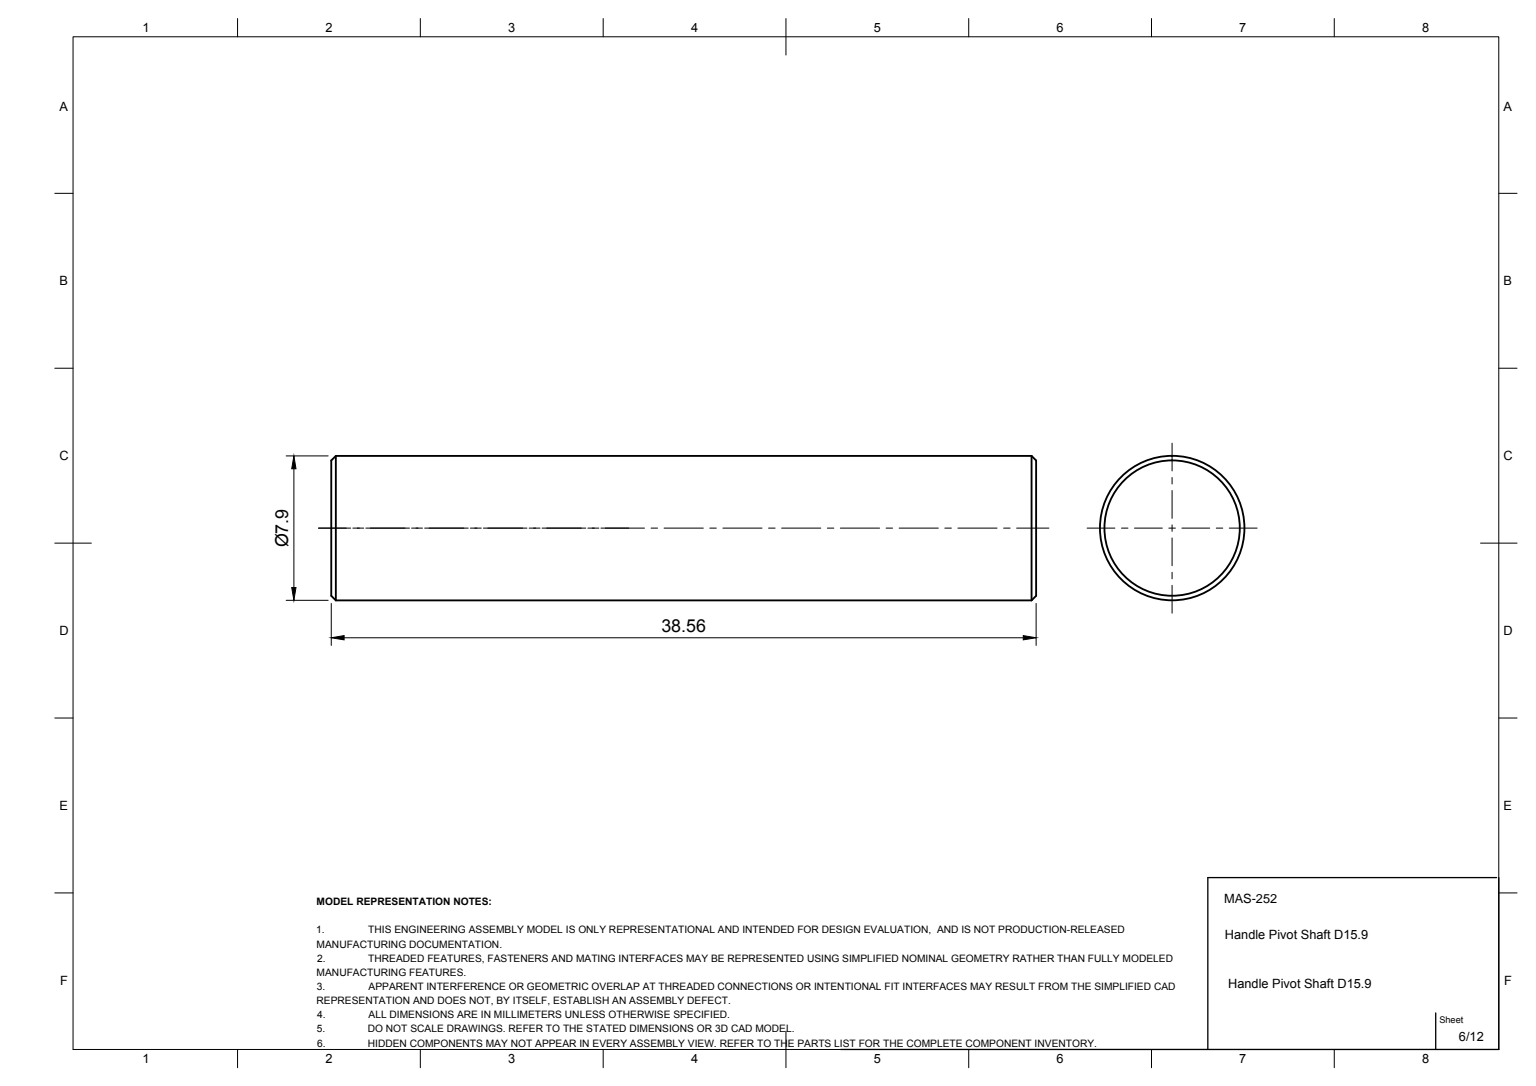
ISO-10303-21;
HEADER;
FILE_DESCRIPTION((''),'2;1');
FILE_NAME('Handle Pivot Shaft D15.9.step','2026-10-06T07:01:46+05:00',(''),(''),'','','');
FILE_SCHEMA (('AUTOMOTIVE_DESIGN { 1 0 10303 214 3 1 1 }'));
ENDSEC;
DATA;
#10=MECHANICAL_DESIGN_GEOMETRIC_PRESENTATION_REPRESENTATION('',(#141),#11396);
#95=CONICAL_SURFACE('',#6218,3.825,0.785398163397448) ;
#96=CONICAL_SURFACE('',#6222,3.825,0.785398163397448) ;
#111=SHAPE_REPRESENTATION_RELATIONSHIP('SRR','None',#11458,#126) ;
#126=ADVANCED_BREP_SHAPE_REPRESENTATION('',(#156),#11384) ;
#141=STYLED_ITEM('',(#11542),#156) ;
#156=MANIFOLD_SOLID_BREP('Handle Pivot Shaft D15.9',#5572) ;
#460=PLANE('',#6216) ;
#461=PLANE('',#6224) ;
#752=FACE_OUTER_BOUND('',#1114,.T.) ;
#753=FACE_OUTER_BOUND('',#1115,.T.) ;
#754=FACE_OUTER_BOUND('',#1116,.T.) ;
#755=FACE_OUTER_BOUND('',#1117,.T.) ;
#756=FACE_OUTER_BOUND('',#1118,.T.) ;
#1114=EDGE_LOOP('',(#4712)) ;
#1115=EDGE_LOOP('',(#4713,#4714,#4715,#4716)) ;
#1116=EDGE_LOOP('',(#4717,#4718,#4719,#4720)) ;
#1117=EDGE_LOOP('',(#4721,#4722,#4723,#4724)) ;
#1118=EDGE_LOOP('',(#4725)) ;
#1495=LINE('',#10802,#1878) ;
#1496=LINE('',#10806,#1879) ;
#1497=LINE('',#10810,#1880) ;
#1878=VECTOR('',#7629,3.825) ;
#1879=VECTOR('',#7634,3.95) ;
#1880=VECTOR('',#7639,3.825) ;
#2194=CIRCLE('',#6217,3.7) ;
#2195=CIRCLE('',#6219,3.95) ;
#2196=CIRCLE('',#6221,3.95) ;
#2197=CIRCLE('',#6223,3.7) ;
#2623=VERTEX_POINT('',#10797) ;
#2624=VERTEX_POINT('',#10800) ;
#2625=VERTEX_POINT('',#10804) ;
#2626=VERTEX_POINT('',#10808) ;
#3338=EDGE_CURVE('',#2623,#2623,#2194,.T.) ;
#3339=EDGE_CURVE('',#2624,#2624,#2195,.T.) ;
#3340=EDGE_CURVE('',#2624,#2623,#1495,.T.) ;
#3341=EDGE_CURVE('',#2625,#2625,#2196,.T.) ;
#3342=EDGE_CURVE('',#2625,#2624,#1496,.T.) ;
#3343=EDGE_CURVE('',#2626,#2626,#2197,.T.) ;
#3344=EDGE_CURVE('',#2626,#2625,#1497,.T.) ;
#4712=ORIENTED_EDGE('',*,*,#3338,.F.) ;
#4713=ORIENTED_EDGE('',*,*,#3339,.F.) ;
#4714=ORIENTED_EDGE('',*,*,#3340,.T.) ;
#4715=ORIENTED_EDGE('',*,*,#3338,.T.) ;
#4716=ORIENTED_EDGE('',*,*,#3340,.F.) ;
#4717=ORIENTED_EDGE('',*,*,#3341,.F.) ;
#4718=ORIENTED_EDGE('',*,*,#3342,.T.) ;
#4719=ORIENTED_EDGE('',*,*,#3339,.T.) ;
#4720=ORIENTED_EDGE('',*,*,#3342,.F.) ;
#4721=ORIENTED_EDGE('',*,*,#3343,.F.) ;
#4722=ORIENTED_EDGE('',*,*,#3344,.T.) ;
#4723=ORIENTED_EDGE('',*,*,#3341,.T.) ;
#4724=ORIENTED_EDGE('',*,*,#3344,.F.) ;
#4725=ORIENTED_EDGE('',*,*,#3343,.T.) ;
#5204=CYLINDRICAL_SURFACE('',#6220,3.95) ;
#5477=ADVANCED_FACE('',(#752),#460,.T.) ;
#5478=ADVANCED_FACE('',(#753),#95,.T.) ;
#5479=ADVANCED_FACE('',(#754),#5204,.T.) ;
#5480=ADVANCED_FACE('',(#755),#96,.T.) ;
#5481=ADVANCED_FACE('',(#756),#461,.T.) ;
#5572=CLOSED_SHELL('',(#5477,#5478,#5479,#5480,#5481)) ;
#6215=AXIS2_PLACEMENT_3D('',#10795,#7619,#7620) ;
#6216=AXIS2_PLACEMENT_3D('',#10796,#7621,#7622) ;
#6217=AXIS2_PLACEMENT_3D('',#10798,#7623,#7624) ;
#6218=AXIS2_PLACEMENT_3D('',#10799,#7625,#7626) ;
#6219=AXIS2_PLACEMENT_3D('',#10801,#7627,#7628) ;
#6220=AXIS2_PLACEMENT_3D('',#10803,#7630,#7631) ;
#6221=AXIS2_PLACEMENT_3D('',#10805,#7632,#7633) ;
#6222=AXIS2_PLACEMENT_3D('',#10807,#7635,#7636) ;
#6223=AXIS2_PLACEMENT_3D('',#10809,#7637,#7638) ;
#6224=AXIS2_PLACEMENT_3D('',#10811,#7640,#7641) ;
#7619=DIRECTION('axis',(0.,0.,1.)) ;
#7620=DIRECTION('refdir',(1.,0.,0.)) ;
#7621=DIRECTION('center_axis',(-1.,0.,0.)) ;
#7622=DIRECTION('ref_axis',(0.,0.,1.)) ;
#7623=DIRECTION('center_axis',(1.,0.,0.)) ;
#7624=DIRECTION('ref_axis',(0.,0.,-1.)) ;
#7625=DIRECTION('center_axis',(1.,0.,0.)) ;
#7626=DIRECTION('ref_axis',(0.,1.,0.)) ;
#7627=DIRECTION('center_axis',(1.,0.,0.)) ;
#7628=DIRECTION('ref_axis',(0.,0.,-1.)) ;
#7629=DIRECTION('',(-0.707106781186548,0.707106781186548,8.65956056235493E-17)) ;
#7630=DIRECTION('center_axis',(1.,0.,0.)) ;
#7631=DIRECTION('ref_axis',(0.,1.,0.)) ;
#7632=DIRECTION('center_axis',(1.,0.,0.)) ;
#7633=DIRECTION('ref_axis',(0.,0.,-1.)) ;
#7634=DIRECTION('',(-1.,0.,0.)) ;
#7635=DIRECTION('center_axis',(-1.,0.,0.)) ;
#7636=DIRECTION('ref_axis',(0.,1.,0.)) ;
#7637=DIRECTION('center_axis',(1.,0.,0.)) ;
#7638=DIRECTION('ref_axis',(0.,0.,-1.)) ;
#7639=DIRECTION('',(-0.707106781186548,-0.707106781186548,-8.65956056235493E-17)) ;
#7640=DIRECTION('center_axis',(1.,0.,0.)) ;
#7641=DIRECTION('ref_axis',(0.,0.,-1.)) ;
#10795=CARTESIAN_POINT('',(0.,0.,0.)) ;
#10796=CARTESIAN_POINT('Origin',(-27.15,21.265,27.14)) ;
#10797=CARTESIAN_POINT('',(-27.15,13.865,27.14)) ;
#10798=CARTESIAN_POINT('Origin',(-27.15,17.565,27.14)) ;
#10799=CARTESIAN_POINT('Origin',(-27.025,17.565,27.14)) ;
#10800=CARTESIAN_POINT('',(-26.9,13.615,27.14)) ;
#10801=CARTESIAN_POINT('Origin',(-26.9,17.565,27.14)) ;
#10802=CARTESIAN_POINT('',(-27.025,13.74,27.14)) ;
#10803=CARTESIAN_POINT('Origin',(-7.87,17.565,27.14)) ;
#10804=CARTESIAN_POINT('',(11.16,13.615,27.14)) ;
#10805=CARTESIAN_POINT('Origin',(11.16,17.565,27.14)) ;
#10806=CARTESIAN_POINT('',(-7.87,13.615,27.14)) ;
#10807=CARTESIAN_POINT('Origin',(11.285,17.565,27.14)) ;
#10808=CARTESIAN_POINT('',(11.41,13.865,27.14)) ;
#10809=CARTESIAN_POINT('Origin',(11.41,17.565,27.14)) ;
#10810=CARTESIAN_POINT('',(11.285,13.74,27.14)) ;
#10811=CARTESIAN_POINT('Origin',(11.41,17.565,27.14)) ;
#11367=UNCERTAINTY_MEASURE_WITH_UNIT(LENGTH_MEASURE(0.01),#11397,
'DISTANCE_ACCURACY_VALUE',
'Maximum model space distance between geometric entities at asserted c
onnectivities') ;
#11379=UNCERTAINTY_MEASURE_WITH_UNIT(LENGTH_MEASURE(0.01),#11397,
'DISTANCE_ACCURACY_VALUE',
'Maximum model space distance between geometric entities at asserted c
onnectivities') ;
#11384=(
GEOMETRIC_REPRESENTATION_CONTEXT(3)
GLOBAL_UNCERTAINTY_ASSIGNED_CONTEXT((#11367))
GLOBAL_UNIT_ASSIGNED_CONTEXT((#11397,#11399,#11400))
REPRESENTATION_CONTEXT('','3D')
) ;
#11396=(
GEOMETRIC_REPRESENTATION_CONTEXT(3)
GLOBAL_UNCERTAINTY_ASSIGNED_CONTEXT((#11379))
GLOBAL_UNIT_ASSIGNED_CONTEXT((#11397,#11399,#11400))
REPRESENTATION_CONTEXT('','3D')
) ;
#11397=(
LENGTH_UNIT()
NAMED_UNIT(*)
SI_UNIT(.MILLI.,.METRE.)
) ;
#11399=(
NAMED_UNIT(*)
PLANE_ANGLE_UNIT()
SI_UNIT($,.RADIAN.)
) ;
#11400=(
NAMED_UNIT(*)
SI_UNIT($,.STERADIAN.)
SOLID_ANGLE_UNIT()
) ;
#11405=SHAPE_DEFINITION_REPRESENTATION(#11421,#11458) ;
#11421=PRODUCT_DEFINITION_SHAPE('',$,#11475) ;
#11458=SHAPE_REPRESENTATION('',(#6215),#11384) ;
#11470=PRODUCT_DEFINITION_CONTEXT('part definition',#11520,'design') ;
#11475=PRODUCT_DEFINITION('Handle Pivot Shaft D15.9',
'Handle Pivot Shaft D15.9',#11491,#11470) ;
#11491=PRODUCT_DEFINITION_FORMATION('',$,#11526) ;
#11520=APPLICATION_CONTEXT(
'Core Data for Automotive Mechanical Design Process') ;
#11521=PRODUCT_CONTEXT('part definition',#11520,'mechanical') ;
#11526=PRODUCT('Handle Pivot Shaft D15.9','Handle Pivot Shaft D15.9',$,(#11521)) ;
#11542=PRESENTATION_STYLE_ASSIGNMENT((#11558)) ;
#11558=SURFACE_STYLE_USAGE(.BOTH.,#11574) ;
#11574=SURFACE_SIDE_STYLE('',(#11590)) ;
#11590=SURFACE_STYLE_FILL_AREA(#11606) ;
#11606=FILL_AREA_STYLE('MAS-252 Metallic - Handle Pivot Shaft D15.9',(#11622)) ;
#11622=FILL_AREA_STYLE_COLOUR(
'MAS-252 Metallic - Handle Pivot Shaft D15.9',#11638) ;
#11638=COLOUR_RGB('MAS-252 Metallic - Handle Pivot Shaft D15.9', 0.40784314, 0.44705882, 0.49803922) ;
ENDSEC;
END-ISO-10303-21;
